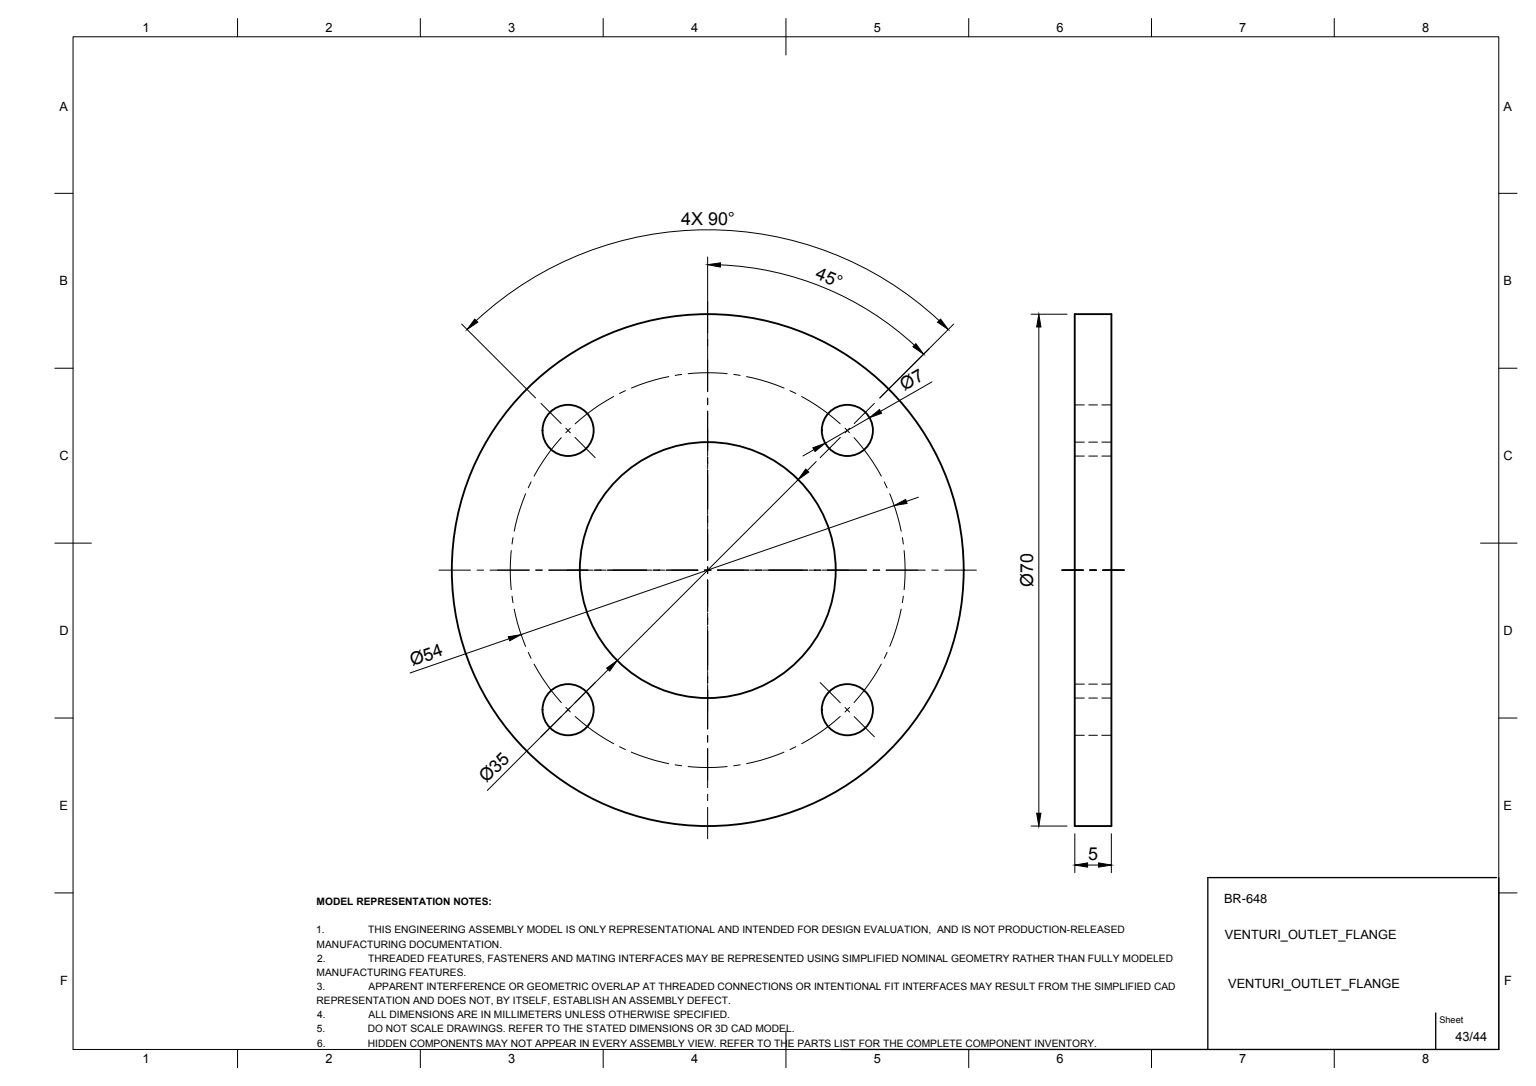
ISO-10303-21;
HEADER;
FILE_DESCRIPTION((''),'2;1');
FILE_NAME('VENTURI_OUTLET_FLANGE.step','2026-10-01T22:05:39-07:00',(''),(''),'','','');
FILE_SCHEMA (('AUTOMOTIVE_DESIGN { 1 0 10303 214 3 1 1 }'));
ENDSEC;
DATA;
#10=MECHANICAL_DESIGN_GEOMETRIC_PRESENTATION_REPRESENTATION('',(#639),#24628);
#555=SHAPE_REPRESENTATION_RELATIONSHIP('SRR','None',#24829,#597) ;
#597=ADVANCED_BREP_SHAPE_REPRESENTATION('',(#678),#24619) ;
#639=STYLED_ITEM('',(#25031),#678) ;
#678=MANIFOLD_SOLID_BREP('VENTURI_OUTLET_FLANGE',#13181) ;
#924=FACE_BOUND('',#4661,.T.) ;
#925=FACE_BOUND('',#4662,.T.) ;
#926=FACE_BOUND('',#4663,.T.) ;
#927=FACE_BOUND('',#4664,.T.) ;
#928=FACE_BOUND('',#4665,.T.) ;
#929=FACE_BOUND('',#4667,.T.) ;
#930=FACE_BOUND('',#4668,.T.) ;
#931=FACE_BOUND('',#4669,.T.) ;
#932=FACE_BOUND('',#4670,.T.) ;
#933=FACE_BOUND('',#4671,.T.) ;
#1730=LINE('',#24149,#2566) ;
#1731=LINE('',#24155,#2567) ;
#1732=LINE('',#24161,#2568) ;
#1733=LINE('',#24167,#2569) ;
#1734=LINE('',#24173,#2570) ;
#1735=LINE('',#24179,#2571) ;
#2566=VECTOR('',#19307,0.35) ;
#2567=VECTOR('',#19314,0.35) ;
#2568=VECTOR('',#19321,0.35) ;
#2569=VECTOR('',#19328,0.35) ;
#2570=VECTOR('',#19335,1.75) ;
#2571=VECTOR('',#19342,3.5) ;
#2932=CYLINDRICAL_SURFACE('',#15244,0.35) ;
#2933=CYLINDRICAL_SURFACE('',#15247,0.35) ;
#2934=CYLINDRICAL_SURFACE('',#15250,0.35) ;
#2935=CYLINDRICAL_SURFACE('',#15253,0.35) ;
#2936=CYLINDRICAL_SURFACE('',#15256,1.75) ;
#2937=CYLINDRICAL_SURFACE('',#15259,3.5) ;
#3649=FACE_OUTER_BOUND('',#4654,.T.) ;
#3650=FACE_OUTER_BOUND('',#4655,.T.) ;
#3651=FACE_OUTER_BOUND('',#4656,.T.) ;
#3652=FACE_OUTER_BOUND('',#4657,.T.) ;
#3653=FACE_OUTER_BOUND('',#4658,.T.) ;
#3654=FACE_OUTER_BOUND('',#4659,.T.) ;
#3655=FACE_OUTER_BOUND('',#4660,.T.) ;
#3656=FACE_OUTER_BOUND('',#4666,.T.) ;
#4654=EDGE_LOOP('',(#11701,#11702,#11703,#11704)) ;
#4655=EDGE_LOOP('',(#11705,#11706,#11707,#11708)) ;
#4656=EDGE_LOOP('',(#11709,#11710,#11711,#11712)) ;
#4657=EDGE_LOOP('',(#11713,#11714,#11715,#11716)) ;
#4658=EDGE_LOOP('',(#11717,#11718,#11719,#11720)) ;
#4659=EDGE_LOOP('',(#11721,#11722,#11723,#11724)) ;
#4660=EDGE_LOOP('',(#11725)) ;
#4661=EDGE_LOOP('',(#11726)) ;
#4662=EDGE_LOOP('',(#11727)) ;
#4663=EDGE_LOOP('',(#11728)) ;
#4664=EDGE_LOOP('',(#11729)) ;
#4665=EDGE_LOOP('',(#11730)) ;
#4666=EDGE_LOOP('',(#11731)) ;
#4667=EDGE_LOOP('',(#11732)) ;
#4668=EDGE_LOOP('',(#11733)) ;
#4669=EDGE_LOOP('',(#11734)) ;
#4670=EDGE_LOOP('',(#11735)) ;
#4671=EDGE_LOOP('',(#11736)) ;
#5499=CIRCLE('',#15245,0.35) ;
#5500=CIRCLE('',#15246,0.35) ;
#5501=CIRCLE('',#15248,0.35) ;
#5502=CIRCLE('',#15249,0.35) ;
#5503=CIRCLE('',#15251,0.35) ;
#5504=CIRCLE('',#15252,0.35) ;
#5505=CIRCLE('',#15254,0.35) ;
#5506=CIRCLE('',#15255,0.35) ;
#5507=CIRCLE('',#15257,1.75) ;
#5508=CIRCLE('',#15258,1.75) ;
#5509=CIRCLE('',#15260,3.5) ;
#5510=CIRCLE('',#15261,3.5) ;
#6635=VERTEX_POINT('',#24146) ;
#6636=VERTEX_POINT('',#24148) ;
#6637=VERTEX_POINT('',#24152) ;
#6638=VERTEX_POINT('',#24154) ;
#6639=VERTEX_POINT('',#24158) ;
#6640=VERTEX_POINT('',#24160) ;
#6641=VERTEX_POINT('',#24164) ;
#6642=VERTEX_POINT('',#24166) ;
#6643=VERTEX_POINT('',#24170) ;
#6644=VERTEX_POINT('',#24172) ;
#6645=VERTEX_POINT('',#24176) ;
#6646=VERTEX_POINT('',#24178) ;
#8340=EDGE_CURVE('',#6635,#6635,#5499,.T.) ;
#8341=EDGE_CURVE('',#6635,#6636,#1730,.T.) ;
#8342=EDGE_CURVE('',#6636,#6636,#5500,.T.) ;
#8343=EDGE_CURVE('',#6637,#6637,#5501,.T.) ;
#8344=EDGE_CURVE('',#6637,#6638,#1731,.T.) ;
#8345=EDGE_CURVE('',#6638,#6638,#5502,.T.) ;
#8346=EDGE_CURVE('',#6639,#6639,#5503,.T.) ;
#8347=EDGE_CURVE('',#6639,#6640,#1732,.T.) ;
#8348=EDGE_CURVE('',#6640,#6640,#5504,.T.) ;
#8349=EDGE_CURVE('',#6641,#6641,#5505,.T.) ;
#8350=EDGE_CURVE('',#6641,#6642,#1733,.T.) ;
#8351=EDGE_CURVE('',#6642,#6642,#5506,.T.) ;
#8352=EDGE_CURVE('',#6643,#6643,#5507,.T.) ;
#8353=EDGE_CURVE('',#6643,#6644,#1734,.T.) ;
#8354=EDGE_CURVE('',#6644,#6644,#5508,.T.) ;
#8355=EDGE_CURVE('',#6645,#6645,#5509,.T.) ;
#8356=EDGE_CURVE('',#6645,#6646,#1735,.T.) ;
#8357=EDGE_CURVE('',#6646,#6646,#5510,.T.) ;
#11701=ORIENTED_EDGE('',*,*,#8340,.F.) ;
#11702=ORIENTED_EDGE('',*,*,#8341,.T.) ;
#11703=ORIENTED_EDGE('',*,*,#8342,.F.) ;
#11704=ORIENTED_EDGE('',*,*,#8341,.F.) ;
#11705=ORIENTED_EDGE('',*,*,#8343,.F.) ;
#11706=ORIENTED_EDGE('',*,*,#8344,.T.) ;
#11707=ORIENTED_EDGE('',*,*,#8345,.F.) ;
#11708=ORIENTED_EDGE('',*,*,#8344,.F.) ;
#11709=ORIENTED_EDGE('',*,*,#8346,.F.) ;
#11710=ORIENTED_EDGE('',*,*,#8347,.T.) ;
#11711=ORIENTED_EDGE('',*,*,#8348,.F.) ;
#11712=ORIENTED_EDGE('',*,*,#8347,.F.) ;
#11713=ORIENTED_EDGE('',*,*,#8349,.F.) ;
#11714=ORIENTED_EDGE('',*,*,#8350,.T.) ;
#11715=ORIENTED_EDGE('',*,*,#8351,.F.) ;
#11716=ORIENTED_EDGE('',*,*,#8350,.F.) ;
#11717=ORIENTED_EDGE('',*,*,#8352,.F.) ;
#11718=ORIENTED_EDGE('',*,*,#8353,.T.) ;
#11719=ORIENTED_EDGE('',*,*,#8354,.F.) ;
#11720=ORIENTED_EDGE('',*,*,#8353,.F.) ;
#11721=ORIENTED_EDGE('',*,*,#8355,.F.) ;
#11722=ORIENTED_EDGE('',*,*,#8356,.T.) ;
#11723=ORIENTED_EDGE('',*,*,#8357,.F.) ;
#11724=ORIENTED_EDGE('',*,*,#8356,.F.) ;
#11725=ORIENTED_EDGE('',*,*,#8357,.T.) ;
#11726=ORIENTED_EDGE('',*,*,#8340,.T.) ;
#11727=ORIENTED_EDGE('',*,*,#8343,.T.) ;
#11728=ORIENTED_EDGE('',*,*,#8346,.T.) ;
#11729=ORIENTED_EDGE('',*,*,#8349,.T.) ;
#11730=ORIENTED_EDGE('',*,*,#8352,.T.) ;
#11731=ORIENTED_EDGE('',*,*,#8355,.T.) ;
#11732=ORIENTED_EDGE('',*,*,#8342,.T.) ;
#11733=ORIENTED_EDGE('',*,*,#8345,.T.) ;
#11734=ORIENTED_EDGE('',*,*,#8348,.T.) ;
#11735=ORIENTED_EDGE('',*,*,#8351,.T.) ;
#11736=ORIENTED_EDGE('',*,*,#8354,.T.) ;
#12297=PLANE('',#15262) ;
#12298=PLANE('',#15263) ;
#13044=ADVANCED_FACE('',(#3649),#2932,.F.) ;
#13045=ADVANCED_FACE('',(#3650),#2933,.F.) ;
#13046=ADVANCED_FACE('',(#3651),#2934,.F.) ;
#13047=ADVANCED_FACE('',(#3652),#2935,.F.) ;
#13048=ADVANCED_FACE('',(#3653),#2936,.F.) ;
#13049=ADVANCED_FACE('',(#3654),#2937,.T.) ;
#13050=ADVANCED_FACE('',(#3655,#924,#925,#926,#927,#928),#12297,.T.) ;
#13051=ADVANCED_FACE('',(#3656,#929,#930,#931,#932,#933),#12298,.T.) ;
#13181=CLOSED_SHELL('',(#13044,#13045,#13046,#13047,#13048,#13049,#13050,
#13051)) ;
#15243=AXIS2_PLACEMENT_3D('',#24144,#19301,#19302) ;
#15244=AXIS2_PLACEMENT_3D('',#24145,#19303,#19304) ;
#15245=AXIS2_PLACEMENT_3D('',#24147,#19305,#19306) ;
#15246=AXIS2_PLACEMENT_3D('',#24150,#19308,#19309) ;
#15247=AXIS2_PLACEMENT_3D('',#24151,#19310,#19311) ;
#15248=AXIS2_PLACEMENT_3D('',#24153,#19312,#19313) ;
#15249=AXIS2_PLACEMENT_3D('',#24156,#19315,#19316) ;
#15250=AXIS2_PLACEMENT_3D('',#24157,#19317,#19318) ;
#15251=AXIS2_PLACEMENT_3D('',#24159,#19319,#19320) ;
#15252=AXIS2_PLACEMENT_3D('',#24162,#19322,#19323) ;
#15253=AXIS2_PLACEMENT_3D('',#24163,#19324,#19325) ;
#15254=AXIS2_PLACEMENT_3D('',#24165,#19326,#19327) ;
#15255=AXIS2_PLACEMENT_3D('',#24168,#19329,#19330) ;
#15256=AXIS2_PLACEMENT_3D('',#24169,#19331,#19332) ;
#15257=AXIS2_PLACEMENT_3D('',#24171,#19333,#19334) ;
#15258=AXIS2_PLACEMENT_3D('',#24174,#19336,#19337) ;
#15259=AXIS2_PLACEMENT_3D('',#24175,#19338,#19339) ;
#15260=AXIS2_PLACEMENT_3D('',#24177,#19340,#19341) ;
#15261=AXIS2_PLACEMENT_3D('',#24180,#19343,#19344) ;
#15262=AXIS2_PLACEMENT_3D('',#24181,#19345,#19346) ;
#15263=AXIS2_PLACEMENT_3D('',#24182,#19347,#19348) ;
#19301=DIRECTION('axis',(0.,0.,1.)) ;
#19302=DIRECTION('refdir',(1.,0.,0.)) ;
#19303=DIRECTION('center_axis',(1.,0.,0.)) ;
#19304=DIRECTION('ref_axis',(0.,0.,-1.)) ;
#19305=DIRECTION('center_axis',(1.,0.,0.)) ;
#19306=DIRECTION('ref_axis',(0.,0.,-1.)) ;
#19307=DIRECTION('',(1.,0.,0.)) ;
#19308=DIRECTION('center_axis',(-1.,0.,0.)) ;
#19309=DIRECTION('ref_axis',(0.,0.,-1.)) ;
#19310=DIRECTION('center_axis',(1.,0.,0.)) ;
#19311=DIRECTION('ref_axis',(0.,0.,-1.)) ;
#19312=DIRECTION('center_axis',(1.,0.,0.)) ;
#19313=DIRECTION('ref_axis',(0.,0.,-1.)) ;
#19314=DIRECTION('',(1.,0.,0.)) ;
#19315=DIRECTION('center_axis',(-1.,0.,0.)) ;
#19316=DIRECTION('ref_axis',(0.,0.,-1.)) ;
#19317=DIRECTION('center_axis',(1.,0.,0.)) ;
#19318=DIRECTION('ref_axis',(0.,0.,-1.)) ;
#19319=DIRECTION('center_axis',(1.,0.,0.)) ;
#19320=DIRECTION('ref_axis',(0.,0.,-1.)) ;
#19321=DIRECTION('',(1.,0.,0.)) ;
#19322=DIRECTION('center_axis',(-1.,0.,0.)) ;
#19323=DIRECTION('ref_axis',(0.,0.,-1.)) ;
#19324=DIRECTION('center_axis',(1.,0.,0.)) ;
#19325=DIRECTION('ref_axis',(0.,0.,-1.)) ;
#19326=DIRECTION('center_axis',(1.,0.,0.)) ;
#19327=DIRECTION('ref_axis',(0.,0.,-1.)) ;
#19328=DIRECTION('',(1.,0.,0.)) ;
#19329=DIRECTION('center_axis',(-1.,0.,0.)) ;
#19330=DIRECTION('ref_axis',(0.,0.,-1.)) ;
#19331=DIRECTION('center_axis',(1.,0.,0.)) ;
#19332=DIRECTION('ref_axis',(0.,0.,-1.)) ;
#19333=DIRECTION('center_axis',(1.,0.,0.)) ;
#19334=DIRECTION('ref_axis',(0.,0.,-1.)) ;
#19335=DIRECTION('',(1.,0.,0.)) ;
#19336=DIRECTION('center_axis',(-1.,0.,0.)) ;
#19337=DIRECTION('ref_axis',(0.,0.,-1.)) ;
#19338=DIRECTION('center_axis',(1.,0.,0.)) ;
#19339=DIRECTION('ref_axis',(0.,0.,-1.)) ;
#19340=DIRECTION('center_axis',(1.,0.,0.)) ;
#19341=DIRECTION('ref_axis',(0.,0.,-1.)) ;
#19342=DIRECTION('',(-1.,0.,0.)) ;
#19343=DIRECTION('center_axis',(-1.,0.,0.)) ;
#19344=DIRECTION('ref_axis',(0.,0.,-1.)) ;
#19345=DIRECTION('center_axis',(-1.,0.,0.)) ;
#19346=DIRECTION('ref_axis',(0.,0.,1.)) ;
#19347=DIRECTION('center_axis',(1.,0.,0.)) ;
#19348=DIRECTION('ref_axis',(0.,0.,-1.)) ;
#24144=CARTESIAN_POINT('',(0.,0.,0.)) ;
#24145=CARTESIAN_POINT('Origin',(7.75,0.109188309203678,-18.4091883092037)) ;
#24146=CARTESIAN_POINT('',(7.5,0.109188309203678,-18.0591883092037)) ;
#24147=CARTESIAN_POINT('Origin',(7.5,0.109188309203678,-18.4091883092037)) ;
#24148=CARTESIAN_POINT('',(8.,0.109188309203678,-18.0591883092037)) ;
#24149=CARTESIAN_POINT('',(7.75,0.109188309203678,-18.0591883092037)) ;
#24150=CARTESIAN_POINT('Origin',(8.,0.109188309203678,-18.4091883092037)) ;
#24151=CARTESIAN_POINT('Origin',(7.75,-3.70918830920368,-18.4091883092037)) ;
#24152=CARTESIAN_POINT('',(7.5,-3.70918830920368,-18.0591883092037)) ;
#24153=CARTESIAN_POINT('Origin',(7.5,-3.70918830920368,-18.4091883092037)) ;
#24154=CARTESIAN_POINT('',(8.,-3.70918830920368,-18.0591883092037)) ;
#24155=CARTESIAN_POINT('',(7.75,-3.70918830920368,-18.0591883092037)) ;
#24156=CARTESIAN_POINT('Origin',(8.,-3.70918830920368,-18.4091883092037)) ;
#24157=CARTESIAN_POINT('Origin',(7.75,-3.70918830920368,-14.5908116907963)) ;
#24158=CARTESIAN_POINT('',(7.5,-3.70918830920368,-14.2408116907963)) ;
#24159=CARTESIAN_POINT('Origin',(7.5,-3.70918830920368,-14.5908116907963)) ;
#24160=CARTESIAN_POINT('',(8.,-3.70918830920368,-14.2408116907963)) ;
#24161=CARTESIAN_POINT('',(7.75,-3.70918830920368,-14.2408116907963)) ;
#24162=CARTESIAN_POINT('Origin',(8.,-3.70918830920368,-14.5908116907963)) ;
#24163=CARTESIAN_POINT('Origin',(7.75,0.109188309203678,-14.5908116907963)) ;
#24164=CARTESIAN_POINT('',(7.5,0.109188309203678,-14.2408116907963)) ;
#24165=CARTESIAN_POINT('Origin',(7.5,0.109188309203678,-14.5908116907963)) ;
#24166=CARTESIAN_POINT('',(8.,0.109188309203679,-14.2408116907963)) ;
#24167=CARTESIAN_POINT('',(7.75,0.109188309203678,-14.2408116907963)) ;
#24168=CARTESIAN_POINT('Origin',(8.,0.109188309203678,-14.5908116907963)) ;
#24169=CARTESIAN_POINT('Origin',(7.75,-1.8,-16.5)) ;
#24170=CARTESIAN_POINT('',(7.5,-1.8,-14.75)) ;
#24171=CARTESIAN_POINT('Origin',(7.5,-1.8,-16.5)) ;
#24172=CARTESIAN_POINT('',(8.,-1.8,-14.75)) ;
#24173=CARTESIAN_POINT('',(7.75,-1.8,-14.75)) ;
#24174=CARTESIAN_POINT('Origin',(8.,-1.8,-16.5)) ;
#24175=CARTESIAN_POINT('Origin',(7.75,-1.8,-16.5)) ;
#24176=CARTESIAN_POINT('',(8.,-1.8,-13.)) ;
#24177=CARTESIAN_POINT('Origin',(8.,-1.8,-16.5)) ;
#24178=CARTESIAN_POINT('',(7.5,-1.8,-13.)) ;
#24179=CARTESIAN_POINT('',(7.75,-1.8,-13.)) ;
#24180=CARTESIAN_POINT('Origin',(7.5,-1.8,-16.5)) ;
#24181=CARTESIAN_POINT('Origin',(7.5,-1.8,-16.5)) ;
#24182=CARTESIAN_POINT('Origin',(8.,-1.8,-16.5)) ;
#24571=UNCERTAINTY_MEASURE_WITH_UNIT(LENGTH_MEASURE(0.001),#24629,
'DISTANCE_ACCURACY_VALUE',
'Maximum model space distance between geometric entities at asserted c
onnectivities') ;
#24580=UNCERTAINTY_MEASURE_WITH_UNIT(LENGTH_MEASURE(0.001),#24629,
'DISTANCE_ACCURACY_VALUE',
'Maximum model space distance between geometric entities at asserted c
onnectivities') ;
#24619=(
GEOMETRIC_REPRESENTATION_CONTEXT(3)
GLOBAL_UNCERTAINTY_ASSIGNED_CONTEXT((#24571))
GLOBAL_UNIT_ASSIGNED_CONTEXT((#24629,#24631,#24632))
REPRESENTATION_CONTEXT('','3D')
) ;
#24628=(
GEOMETRIC_REPRESENTATION_CONTEXT(3)
GLOBAL_UNCERTAINTY_ASSIGNED_CONTEXT((#24580))
GLOBAL_UNIT_ASSIGNED_CONTEXT((#24629,#24631,#24632))
REPRESENTATION_CONTEXT('','3D')
) ;
#24629=(
LENGTH_UNIT()
NAMED_UNIT(*)
SI_UNIT(.CENTI.,.METRE.)
) ;
#24631=(
NAMED_UNIT(*)
PLANE_ANGLE_UNIT()
SI_UNIT($,.RADIAN.)
) ;
#24632=(
NAMED_UNIT(*)
SI_UNIT($,.STERADIAN.)
SOLID_ANGLE_UNIT()
) ;
#24671=SHAPE_DEFINITION_REPRESENTATION(#24752,#24829) ;
#24752=PRODUCT_DEFINITION_SHAPE('',$,#24877) ;
#24829=SHAPE_REPRESENTATION('',(#15243),#24619) ;
#24838=PRODUCT_DEFINITION_CONTEXT('part definition',#24981,'design') ;
#24877=PRODUCT_DEFINITION('VENTURI_OUTLET_FLANGE',
'VENTURI_OUTLET_FLANGE',#24924,#24838) ;
#24924=PRODUCT_DEFINITION_FORMATION('',$,#25021) ;
#24981=APPLICATION_CONTEXT(
'Core Data for Automotive Mechanical Design Process') ;
#24982=PRODUCT_CONTEXT('part definition',#24981,'mechanical') ;
#25021=PRODUCT('VENTURI_OUTLET_FLANGE','VENTURI_OUTLET_FLANGE',$,(#24982)) ;
#25031=PRESENTATION_STYLE_ASSIGNMENT((#25041)) ;
#25041=SURFACE_STYLE_USAGE(.BOTH.,#25051) ;
#25051=SURFACE_SIDE_STYLE('',(#25061)) ;
#25061=SURFACE_STYLE_FILL_AREA(#25071) ;
#25071=FILL_AREA_STYLE('Aluminum - Satin',(#25081)) ;
#25081=FILL_AREA_STYLE_COLOUR('Aluminum - Satin',#25091) ;
#25091=COLOUR_RGB('Aluminum - Satin', 0.40784314, 0.44705882, 0.49803922) ;
ENDSEC;
END-ISO-10303-21;
